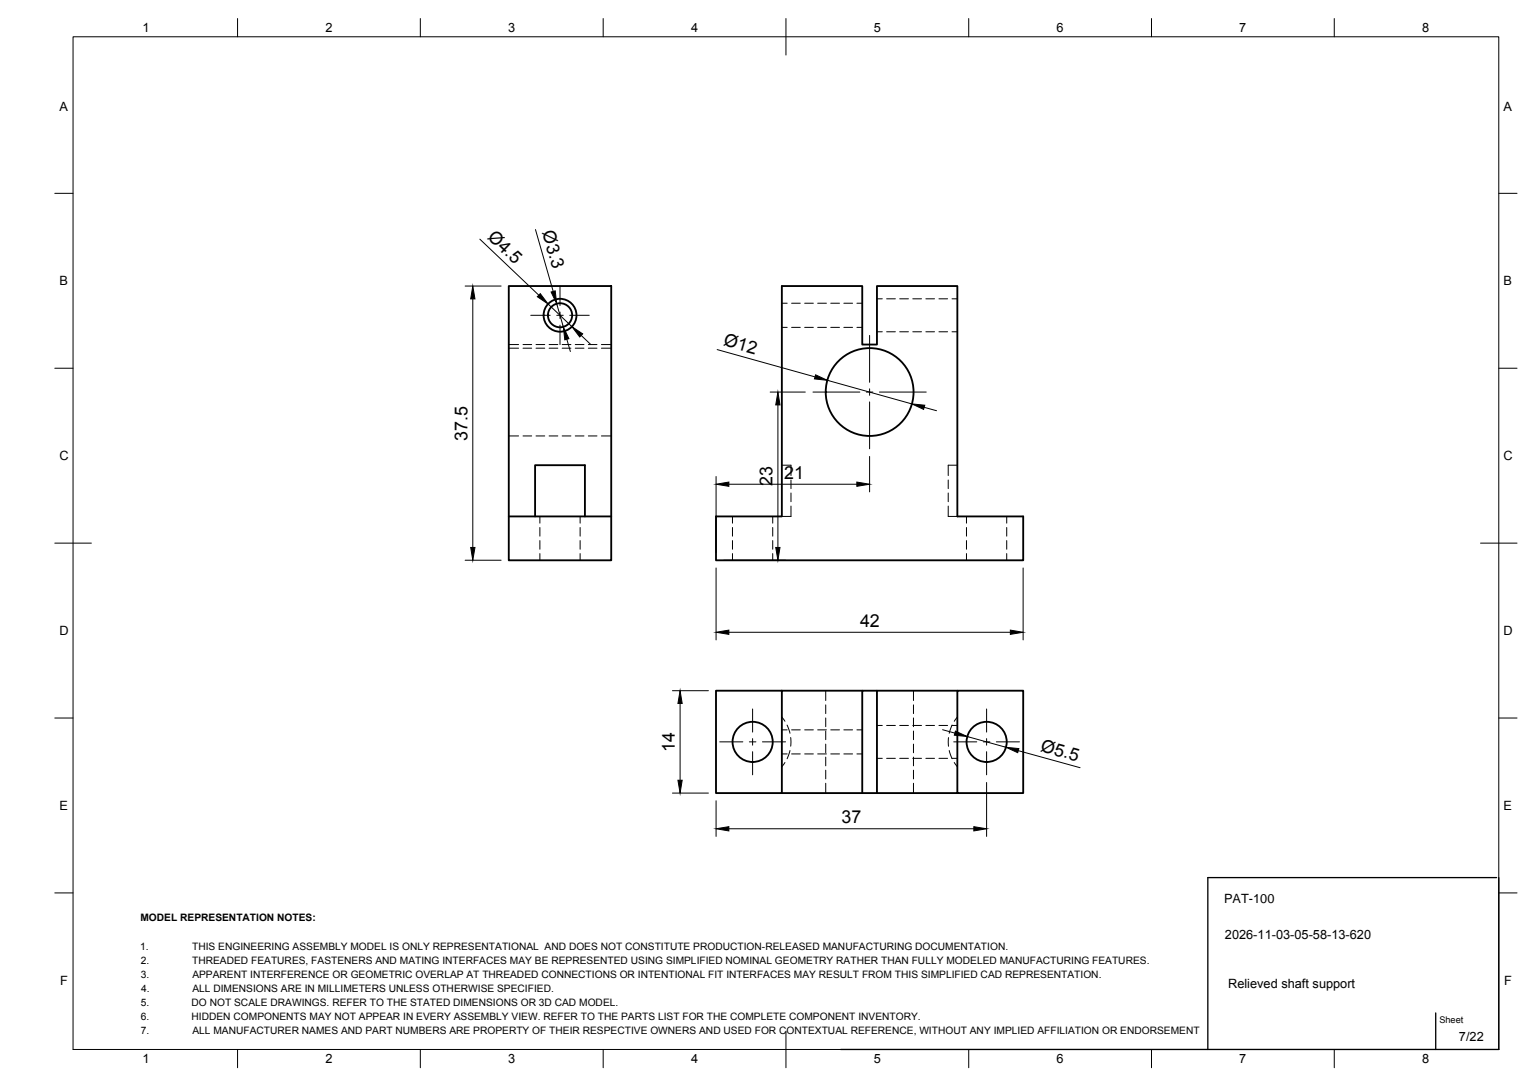
ISO-10303-21;
HEADER;
/* Generated by software containing ST-Developer
 * from STEP Tools, Inc. (www.steptools.com) 
 */

FILE_DESCRIPTION(
/* description */ (''),
/* implementation_level */ '2;1');

FILE_NAME(
/* name */ 'Relieved shaft support.step',
/* time_stamp */ '2026-10-29T16:43:51-07:00',
/* author */ (''),
/* organization */ (''),
/* preprocessor_version */ 'ST-DEVELOPER v20.2',
/* originating_system */ 'Autodesk Translation Framework v15.17.0.0',
/* authorisation */ '');

FILE_SCHEMA (('AUTOMOTIVE_DESIGN { 1 0 10303 214 3 1 1 }'));
ENDSEC;

DATA;
#10=MECHANICAL_DESIGN_GEOMETRIC_PRESENTATION_REPRESENTATION('',(#367),#10292);
#321=SHAPE_REPRESENTATION_RELATIONSHIP('SRR','None',#10417,#344);
#344=ADVANCED_BREP_SHAPE_REPRESENTATION('',(#390),#10269);
#367=STYLED_ITEM('',(#10628),#390);
#390=MANIFOLD_SOLID_BREP('Body1',#5009);
#438=FACE_BOUND('',#1062,.T.);
#439=FACE_BOUND('',#1064,.T.);
#440=FACE_BOUND('',#1066,.T.);
#441=FACE_BOUND('',#1073,.T.);
#442=FACE_BOUND('',#1076,.T.);
#443=FACE_BOUND('',#1077,.T.);
#444=FACE_BOUND('',#1080,.T.);
#445=FACE_BOUND('',#1083,.T.);
#446=FACE_BOUND('',#1086,.T.);
#447=FACE_BOUND('',#1089,.T.);
#539=PLANE('',#5357);
#540=PLANE('',#5364);
#541=PLANE('',#5365);
#542=PLANE('',#5367);
#543=PLANE('',#5369);
#544=PLANE('',#5383);
#545=PLANE('',#5384);
#546=PLANE('',#5385);
#547=PLANE('',#5386);
#548=PLANE('',#5387);
#549=PLANE('',#5388);
#550=PLANE('',#5389);
#551=PLANE('',#5390);
#552=PLANE('',#5391);
#553=PLANE('',#5392);
#554=PLANE('',#5393);
#737=FACE_OUTER_BOUND('',#1057,.T.);
#738=FACE_OUTER_BOUND('',#1058,.T.);
#739=FACE_OUTER_BOUND('',#1059,.T.);
#740=FACE_OUTER_BOUND('',#1060,.T.);
#741=FACE_OUTER_BOUND('',#1061,.T.);
#742=FACE_OUTER_BOUND('',#1063,.T.);
#743=FACE_OUTER_BOUND('',#1065,.T.);
#744=FACE_OUTER_BOUND('',#1067,.T.);
#745=FACE_OUTER_BOUND('',#1068,.T.);
#746=FACE_OUTER_BOUND('',#1069,.T.);
#747=FACE_OUTER_BOUND('',#1070,.T.);
#748=FACE_OUTER_BOUND('',#1071,.T.);
#749=FACE_OUTER_BOUND('',#1072,.T.);
#750=FACE_OUTER_BOUND('',#1074,.T.);
#751=FACE_OUTER_BOUND('',#1075,.T.);
#752=FACE_OUTER_BOUND('',#1078,.T.);
#753=FACE_OUTER_BOUND('',#1079,.T.);
#754=FACE_OUTER_BOUND('',#1081,.T.);
#755=FACE_OUTER_BOUND('',#1082,.T.);
#756=FACE_OUTER_BOUND('',#1084,.T.);
#757=FACE_OUTER_BOUND('',#1085,.T.);
#758=FACE_OUTER_BOUND('',#1087,.T.);
#759=FACE_OUTER_BOUND('',#1088,.T.);
#1057=EDGE_LOOP('',(#3543,#3544));
#1058=EDGE_LOOP('',(#3545,#3546,#3547,#3548));
#1059=EDGE_LOOP('',(#3549,#3550,#3551,#3552));
#1060=EDGE_LOOP('',(#3553,#3554));
#1061=EDGE_LOOP('',(#3555,#3556,#3557,#3558,#3559,#3560));
#1062=EDGE_LOOP('',(#3561));
#1063=EDGE_LOOP('',(#3562,#3563,#3564,#3565,#3566,#3567,#3568,#3569));
#1064=EDGE_LOOP('',(#3570));
#1065=EDGE_LOOP('',(#3571,#3572,#3573,#3574,#3575,#3576));
#1066=EDGE_LOOP('',(#3577));
#1067=EDGE_LOOP('',(#3578,#3579,#3580,#3581));
#1068=EDGE_LOOP('',(#3582,#3583,#3584,#3585));
#1069=EDGE_LOOP('',(#3586,#3587,#3588,#3589));
#1070=EDGE_LOOP('',(#3590,#3591,#3592,#3593));
#1071=EDGE_LOOP('',(#3594,#3595,#3596,#3597));
#1072=EDGE_LOOP('',(#3598,#3599,#3600,#3601,#3602,#3603,#3604,#3605,#3606,
#3607,#3608,#3609));
#1073=EDGE_LOOP('',(#3610));
#1074=EDGE_LOOP('',(#3611,#3612,#3613,#3614));
#1075=EDGE_LOOP('',(#3615,#3616,#3617,#3618));
#1076=EDGE_LOOP('',(#3619));
#1077=EDGE_LOOP('',(#3620));
#1078=EDGE_LOOP('',(#3621,#3622,#3623,#3624));
#1079=EDGE_LOOP('',(#3625,#3626,#3627,#3628,#3629,#3630,#3631,#3632));
#1080=EDGE_LOOP('',(#3633));
#1081=EDGE_LOOP('',(#3634,#3635,#3636,#3637));
#1082=EDGE_LOOP('',(#3638,#3639,#3640,#3641));
#1083=EDGE_LOOP('',(#3642));
#1084=EDGE_LOOP('',(#3643,#3644,#3645,#3646));
#1085=EDGE_LOOP('',(#3647,#3648,#3649,#3650));
#1086=EDGE_LOOP('',(#3651));
#1087=EDGE_LOOP('',(#3652,#3653,#3654,#3655));
#1088=EDGE_LOOP('',(#3656,#3657,#3658,#3659,#3660,#3661,#3662,#3663,#3664,
#3665,#3666,#3667));
#1089=EDGE_LOOP('',(#3668));
#1442=LINE('',#7552,#1834);
#1443=LINE('',#7556,#1835);
#1444=LINE('',#7559,#1836);
#1445=LINE('',#7563,#1837);
#1446=LINE('',#7567,#1838);
#1447=LINE('',#7570,#1839);
#1448=LINE('',#7573,#1840);
#1449=LINE('',#7575,#1841);
#1450=LINE('',#7577,#1842);
#1451=LINE('',#7579,#1843);
#1452=LINE('',#7580,#1844);
#1453=LINE('',#7585,#1845);
#1454=LINE('',#7587,#1846);
#1455=LINE('',#7588,#1847);
#1456=LINE('',#7594,#1848);
#1457=LINE('',#7596,#1849);
#1458=LINE('',#7597,#1850);
#1459=LINE('',#7599,#1851);
#1460=LINE('',#7600,#1852);
#1461=LINE('',#7607,#1853);
#1462=LINE('',#7611,#1854);
#1463=LINE('',#7616,#1855);
#1464=LINE('',#7620,#1856);
#1465=LINE('',#7625,#1857);
#1466=LINE('',#7629,#1858);
#1467=LINE('',#7631,#1859);
#1468=LINE('',#7632,#1860);
#1469=LINE('',#7634,#1861);
#1470=LINE('',#7636,#1862);
#1471=LINE('',#7638,#1863);
#1472=LINE('',#7640,#1864);
#1473=LINE('',#7642,#1865);
#1474=LINE('',#7643,#1866);
#1475=LINE('',#7646,#1867);
#1476=LINE('',#7647,#1868);
#1477=LINE('',#7650,#1869);
#1478=LINE('',#7651,#1870);
#1479=LINE('',#7653,#1871);
#1480=LINE('',#7656,#1872);
#1481=LINE('',#7657,#1873);
#1482=LINE('',#7660,#1874);
#1483=LINE('',#7661,#1875);
#1484=LINE('',#7664,#1876);
#1485=LINE('',#7665,#1877);
#1486=LINE('',#7668,#1878);
#1487=LINE('',#7669,#1879);
#1488=LINE('',#7672,#1880);
#1489=LINE('',#7673,#1881);
#1490=LINE('',#7675,#1882);
#1834=VECTOR('',#6033,1.);
#1835=VECTOR('',#6038,1.);
#1836=VECTOR('',#6041,1.);
#1837=VECTOR('',#6044,1.);
#1838=VECTOR('',#6047,1.);
#1839=VECTOR('',#6052,1.);
#1840=VECTOR('',#6055,1.);
#1841=VECTOR('',#6056,1.);
#1842=VECTOR('',#6057,1.);
#1843=VECTOR('',#6058,1.);
#1844=VECTOR('',#6059,1.);
#1845=VECTOR('',#6064,1.);
#1846=VECTOR('',#6065,1.);
#1847=VECTOR('',#6066,1.);
#1848=VECTOR('',#6071,1.);
#1849=VECTOR('',#6072,1.);
#1850=VECTOR('',#6073,1.);
#1851=VECTOR('',#6074,1.);
#1852=VECTOR('',#6075,1.);
#1853=VECTOR('',#6082,0.225);
#1854=VECTOR('',#6087,0.165);
#1855=VECTOR('',#6094,0.275);
#1856=VECTOR('',#6099,0.275);
#1857=VECTOR('',#6104,0.6);
#1858=VECTOR('',#6109,1.);
#1859=VECTOR('',#6110,1.);
#1860=VECTOR('',#6111,1.);
#1861=VECTOR('',#6112,1.);
#1862=VECTOR('',#6113,1.);
#1863=VECTOR('',#6114,1.);
#1864=VECTOR('',#6115,1.);
#1865=VECTOR('',#6116,1.);
#1866=VECTOR('',#6117,1.);
#1867=VECTOR('',#6120,1.);
#1868=VECTOR('',#6121,1.);
#1869=VECTOR('',#6124,1.);
#1870=VECTOR('',#6125,1.);
#1871=VECTOR('',#6128,1.);
#1872=VECTOR('',#6131,1.);
#1873=VECTOR('',#6132,1.);
#1874=VECTOR('',#6135,1.);
#1875=VECTOR('',#6136,1.);
#1876=VECTOR('',#6139,1.);
#1877=VECTOR('',#6140,1.);
#1878=VECTOR('',#6143,1.);
#1879=VECTOR('',#6144,1.);
#1880=VECTOR('',#6147,1.);
#1881=VECTOR('',#6148,1.);
#1882=VECTOR('',#6151,1.);
#2231=CIRCLE('',#5358,0.525);
#2232=CIRCLE('',#5360,0.525);
#2233=CIRCLE('',#5362,0.525);
#2234=CIRCLE('',#5363,0.525);
#2235=CIRCLE('',#5366,0.275);
#2236=CIRCLE('',#5368,0.165);
#2237=CIRCLE('',#5370,0.275);
#2238=CIRCLE('',#5372,0.225);
#2239=CIRCLE('',#5373,0.225);
#2240=CIRCLE('',#5375,0.165);
#2241=CIRCLE('',#5377,0.275);
#2242=CIRCLE('',#5379,0.275);
#2243=CIRCLE('',#5381,0.6);
#2244=CIRCLE('',#5382,0.6);
#2438=VERTEX_POINT('',#7550);
#2439=VERTEX_POINT('',#7551);
#2440=VERTEX_POINT('',#7555);
#2441=VERTEX_POINT('',#7557);
#2442=VERTEX_POINT('',#7561);
#2443=VERTEX_POINT('',#7562);
#2444=VERTEX_POINT('',#7564);
#2445=VERTEX_POINT('',#7566);
#2446=VERTEX_POINT('',#7572);
#2447=VERTEX_POINT('',#7574);
#2448=VERTEX_POINT('',#7576);
#2449=VERTEX_POINT('',#7578);
#2450=VERTEX_POINT('',#7581);
#2451=VERTEX_POINT('',#7584);
#2452=VERTEX_POINT('',#7586);
#2453=VERTEX_POINT('',#7589);
#2454=VERTEX_POINT('',#7592);
#2455=VERTEX_POINT('',#7593);
#2456=VERTEX_POINT('',#7595);
#2457=VERTEX_POINT('',#7598);
#2458=VERTEX_POINT('',#7601);
#2459=VERTEX_POINT('',#7604);
#2460=VERTEX_POINT('',#7606);
#2461=VERTEX_POINT('',#7610);
#2462=VERTEX_POINT('',#7614);
#2463=VERTEX_POINT('',#7618);
#2464=VERTEX_POINT('',#7622);
#2465=VERTEX_POINT('',#7624);
#2466=VERTEX_POINT('',#7628);
#2467=VERTEX_POINT('',#7630);
#2468=VERTEX_POINT('',#7633);
#2469=VERTEX_POINT('',#7635);
#2470=VERTEX_POINT('',#7637);
#2471=VERTEX_POINT('',#7639);
#2472=VERTEX_POINT('',#7641);
#2473=VERTEX_POINT('',#7645);
#2474=VERTEX_POINT('',#7649);
#2475=VERTEX_POINT('',#7655);
#2476=VERTEX_POINT('',#7659);
#2477=VERTEX_POINT('',#7663);
#2478=VERTEX_POINT('',#7667);
#2479=VERTEX_POINT('',#7671);
#2862=EDGE_CURVE('',#2438,#2439,#1442,.T.);
#2863=EDGE_CURVE('',#2439,#2438,#2231,.T.);
#2864=EDGE_CURVE('',#2440,#2438,#1443,.T.);
#2865=EDGE_CURVE('',#2441,#2440,#2232,.T.);
#2866=EDGE_CURVE('',#2439,#2441,#1444,.T.);
#2867=EDGE_CURVE('',#2442,#2443,#1445,.T.);
#2868=EDGE_CURVE('',#2442,#2444,#2233,.T.);
#2869=EDGE_CURVE('',#2445,#2444,#1446,.T.);
#2870=EDGE_CURVE('',#2443,#2445,#2234,.T.);
#2871=EDGE_CURVE('',#2444,#2442,#1447,.T.);
#2872=EDGE_CURVE('',#2440,#2446,#1448,.T.);
#2873=EDGE_CURVE('',#2447,#2446,#1449,.T.);
#2874=EDGE_CURVE('',#2447,#2448,#1450,.T.);
#2875=EDGE_CURVE('',#2449,#2448,#1451,.T.);
#2876=EDGE_CURVE('',#2449,#2441,#1452,.T.);
#2877=EDGE_CURVE('',#2450,#2450,#2235,.T.);
#2878=EDGE_CURVE('',#2451,#2449,#1453,.T.);
#2879=EDGE_CURVE('',#2451,#2452,#1454,.T.);
#2880=EDGE_CURVE('',#2446,#2452,#1455,.T.);
#2881=EDGE_CURVE('',#2453,#2453,#2236,.T.);
#2882=EDGE_CURVE('',#2454,#2455,#1456,.T.);
#2883=EDGE_CURVE('',#2456,#2455,#1457,.T.);
#2884=EDGE_CURVE('',#2443,#2456,#1458,.T.);
#2885=EDGE_CURVE('',#2457,#2445,#1459,.T.);
#2886=EDGE_CURVE('',#2454,#2457,#1460,.T.);
#2887=EDGE_CURVE('',#2458,#2458,#2237,.T.);
#2888=EDGE_CURVE('',#2459,#2459,#2238,.T.);
#2889=EDGE_CURVE('',#2459,#2460,#1461,.T.);
#2890=EDGE_CURVE('',#2460,#2460,#2239,.T.);
#2891=EDGE_CURVE('',#2453,#2461,#1462,.T.);
#2892=EDGE_CURVE('',#2461,#2461,#2240,.T.);
#2893=EDGE_CURVE('',#2462,#2462,#2241,.T.);
#2894=EDGE_CURVE('',#2462,#2450,#1463,.T.);
#2895=EDGE_CURVE('',#2463,#2463,#2242,.T.);
#2896=EDGE_CURVE('',#2463,#2458,#1464,.T.);
#2897=EDGE_CURVE('',#2464,#2464,#2243,.T.);
#2898=EDGE_CURVE('',#2464,#2465,#1465,.T.);
#2899=EDGE_CURVE('',#2465,#2465,#2244,.T.);
#2900=EDGE_CURVE('',#2448,#2466,#1466,.T.);
#2901=EDGE_CURVE('',#2466,#2467,#1467,.T.);
#2902=EDGE_CURVE('',#2467,#2454,#1468,.T.);
#2903=EDGE_CURVE('',#2457,#2468,#1469,.T.);
#2904=EDGE_CURVE('',#2468,#2469,#1470,.T.);
#2905=EDGE_CURVE('',#2469,#2470,#1471,.T.);
#2906=EDGE_CURVE('',#2470,#2471,#1472,.T.);
#2907=EDGE_CURVE('',#2471,#2472,#1473,.T.);
#2908=EDGE_CURVE('',#2472,#2451,#1474,.T.);
#2909=EDGE_CURVE('',#2473,#2447,#1475,.T.);
#2910=EDGE_CURVE('',#2466,#2473,#1476,.T.);
#2911=EDGE_CURVE('',#2474,#2473,#1477,.T.);
#2912=EDGE_CURVE('',#2467,#2474,#1478,.T.);
#2913=EDGE_CURVE('',#2455,#2474,#1479,.T.);
#2914=EDGE_CURVE('',#2475,#2456,#1480,.T.);
#2915=EDGE_CURVE('',#2468,#2475,#1481,.T.);
#2916=EDGE_CURVE('',#2476,#2475,#1482,.T.);
#2917=EDGE_CURVE('',#2469,#2476,#1483,.T.);
#2918=EDGE_CURVE('',#2477,#2476,#1484,.T.);
#2919=EDGE_CURVE('',#2470,#2477,#1485,.T.);
#2920=EDGE_CURVE('',#2478,#2477,#1486,.T.);
#2921=EDGE_CURVE('',#2471,#2478,#1487,.T.);
#2922=EDGE_CURVE('',#2479,#2478,#1488,.T.);
#2923=EDGE_CURVE('',#2472,#2479,#1489,.T.);
#2924=EDGE_CURVE('',#2452,#2479,#1490,.T.);
#3543=ORIENTED_EDGE('',*,*,#2862,.F.);
#3544=ORIENTED_EDGE('',*,*,#2863,.F.);
#3545=ORIENTED_EDGE('',*,*,#2864,.F.);
#3546=ORIENTED_EDGE('',*,*,#2865,.F.);
#3547=ORIENTED_EDGE('',*,*,#2866,.F.);
#3548=ORIENTED_EDGE('',*,*,#2863,.T.);
#3549=ORIENTED_EDGE('',*,*,#2867,.F.);
#3550=ORIENTED_EDGE('',*,*,#2868,.T.);
#3551=ORIENTED_EDGE('',*,*,#2869,.F.);
#3552=ORIENTED_EDGE('',*,*,#2870,.F.);
#3553=ORIENTED_EDGE('',*,*,#2871,.F.);
#3554=ORIENTED_EDGE('',*,*,#2868,.F.);
#3555=ORIENTED_EDGE('',*,*,#2872,.T.);
#3556=ORIENTED_EDGE('',*,*,#2873,.F.);
#3557=ORIENTED_EDGE('',*,*,#2874,.T.);
#3558=ORIENTED_EDGE('',*,*,#2875,.F.);
#3559=ORIENTED_EDGE('',*,*,#2876,.T.);
#3560=ORIENTED_EDGE('',*,*,#2865,.T.);
#3561=ORIENTED_EDGE('',*,*,#2877,.T.);
#3562=ORIENTED_EDGE('',*,*,#2864,.T.);
#3563=ORIENTED_EDGE('',*,*,#2862,.T.);
#3564=ORIENTED_EDGE('',*,*,#2866,.T.);
#3565=ORIENTED_EDGE('',*,*,#2876,.F.);
#3566=ORIENTED_EDGE('',*,*,#2878,.F.);
#3567=ORIENTED_EDGE('',*,*,#2879,.T.);
#3568=ORIENTED_EDGE('',*,*,#2880,.F.);
#3569=ORIENTED_EDGE('',*,*,#2872,.F.);
#3570=ORIENTED_EDGE('',*,*,#2881,.T.);
#3571=ORIENTED_EDGE('',*,*,#2882,.T.);
#3572=ORIENTED_EDGE('',*,*,#2883,.F.);
#3573=ORIENTED_EDGE('',*,*,#2884,.F.);
#3574=ORIENTED_EDGE('',*,*,#2870,.T.);
#3575=ORIENTED_EDGE('',*,*,#2885,.F.);
#3576=ORIENTED_EDGE('',*,*,#2886,.F.);
#3577=ORIENTED_EDGE('',*,*,#2887,.T.);
#3578=ORIENTED_EDGE('',*,*,#2888,.F.);
#3579=ORIENTED_EDGE('',*,*,#2889,.T.);
#3580=ORIENTED_EDGE('',*,*,#2890,.F.);
#3581=ORIENTED_EDGE('',*,*,#2889,.F.);
#3582=ORIENTED_EDGE('',*,*,#2881,.F.);
#3583=ORIENTED_EDGE('',*,*,#2891,.T.);
#3584=ORIENTED_EDGE('',*,*,#2892,.F.);
#3585=ORIENTED_EDGE('',*,*,#2891,.F.);
#3586=ORIENTED_EDGE('',*,*,#2893,.F.);
#3587=ORIENTED_EDGE('',*,*,#2894,.T.);
#3588=ORIENTED_EDGE('',*,*,#2877,.F.);
#3589=ORIENTED_EDGE('',*,*,#2894,.F.);
#3590=ORIENTED_EDGE('',*,*,#2895,.F.);
#3591=ORIENTED_EDGE('',*,*,#2896,.T.);
#3592=ORIENTED_EDGE('',*,*,#2887,.F.);
#3593=ORIENTED_EDGE('',*,*,#2896,.F.);
#3594=ORIENTED_EDGE('',*,*,#2897,.F.);
#3595=ORIENTED_EDGE('',*,*,#2898,.T.);
#3596=ORIENTED_EDGE('',*,*,#2899,.F.);
#3597=ORIENTED_EDGE('',*,*,#2898,.F.);
#3598=ORIENTED_EDGE('',*,*,#2875,.T.);
#3599=ORIENTED_EDGE('',*,*,#2900,.T.);
#3600=ORIENTED_EDGE('',*,*,#2901,.T.);
#3601=ORIENTED_EDGE('',*,*,#2902,.T.);
#3602=ORIENTED_EDGE('',*,*,#2886,.T.);
#3603=ORIENTED_EDGE('',*,*,#2903,.T.);
#3604=ORIENTED_EDGE('',*,*,#2904,.T.);
#3605=ORIENTED_EDGE('',*,*,#2905,.T.);
#3606=ORIENTED_EDGE('',*,*,#2906,.T.);
#3607=ORIENTED_EDGE('',*,*,#2907,.T.);
#3608=ORIENTED_EDGE('',*,*,#2908,.T.);
#3609=ORIENTED_EDGE('',*,*,#2878,.T.);
#3610=ORIENTED_EDGE('',*,*,#2897,.T.);
#3611=ORIENTED_EDGE('',*,*,#2874,.F.);
#3612=ORIENTED_EDGE('',*,*,#2909,.F.);
#3613=ORIENTED_EDGE('',*,*,#2910,.F.);
#3614=ORIENTED_EDGE('',*,*,#2900,.F.);
#3615=ORIENTED_EDGE('',*,*,#2910,.T.);
#3616=ORIENTED_EDGE('',*,*,#2911,.F.);
#3617=ORIENTED_EDGE('',*,*,#2912,.F.);
#3618=ORIENTED_EDGE('',*,*,#2901,.F.);
#3619=ORIENTED_EDGE('',*,*,#2893,.T.);
#3620=ORIENTED_EDGE('',*,*,#2895,.T.);
#3621=ORIENTED_EDGE('',*,*,#2912,.T.);
#3622=ORIENTED_EDGE('',*,*,#2913,.F.);
#3623=ORIENTED_EDGE('',*,*,#2882,.F.);
#3624=ORIENTED_EDGE('',*,*,#2902,.F.);
#3625=ORIENTED_EDGE('',*,*,#2867,.T.);
#3626=ORIENTED_EDGE('',*,*,#2884,.T.);
#3627=ORIENTED_EDGE('',*,*,#2914,.F.);
#3628=ORIENTED_EDGE('',*,*,#2915,.F.);
#3629=ORIENTED_EDGE('',*,*,#2903,.F.);
#3630=ORIENTED_EDGE('',*,*,#2885,.T.);
#3631=ORIENTED_EDGE('',*,*,#2869,.T.);
#3632=ORIENTED_EDGE('',*,*,#2871,.T.);
#3633=ORIENTED_EDGE('',*,*,#2890,.T.);
#3634=ORIENTED_EDGE('',*,*,#2915,.T.);
#3635=ORIENTED_EDGE('',*,*,#2916,.F.);
#3636=ORIENTED_EDGE('',*,*,#2917,.F.);
#3637=ORIENTED_EDGE('',*,*,#2904,.F.);
#3638=ORIENTED_EDGE('',*,*,#2917,.T.);
#3639=ORIENTED_EDGE('',*,*,#2918,.F.);
#3640=ORIENTED_EDGE('',*,*,#2919,.F.);
#3641=ORIENTED_EDGE('',*,*,#2905,.F.);
#3642=ORIENTED_EDGE('',*,*,#2888,.T.);
#3643=ORIENTED_EDGE('',*,*,#2919,.T.);
#3644=ORIENTED_EDGE('',*,*,#2920,.F.);
#3645=ORIENTED_EDGE('',*,*,#2921,.F.);
#3646=ORIENTED_EDGE('',*,*,#2906,.F.);
#3647=ORIENTED_EDGE('',*,*,#2921,.T.);
#3648=ORIENTED_EDGE('',*,*,#2922,.F.);
#3649=ORIENTED_EDGE('',*,*,#2923,.F.);
#3650=ORIENTED_EDGE('',*,*,#2907,.F.);
#3651=ORIENTED_EDGE('',*,*,#2892,.T.);
#3652=ORIENTED_EDGE('',*,*,#2923,.T.);
#3653=ORIENTED_EDGE('',*,*,#2924,.F.);
#3654=ORIENTED_EDGE('',*,*,#2879,.F.);
#3655=ORIENTED_EDGE('',*,*,#2908,.F.);
#3656=ORIENTED_EDGE('',*,*,#2873,.T.);
#3657=ORIENTED_EDGE('',*,*,#2880,.T.);
#3658=ORIENTED_EDGE('',*,*,#2924,.T.);
#3659=ORIENTED_EDGE('',*,*,#2922,.T.);
#3660=ORIENTED_EDGE('',*,*,#2920,.T.);
#3661=ORIENTED_EDGE('',*,*,#2918,.T.);
#3662=ORIENTED_EDGE('',*,*,#2916,.T.);
#3663=ORIENTED_EDGE('',*,*,#2914,.T.);
#3664=ORIENTED_EDGE('',*,*,#2883,.T.);
#3665=ORIENTED_EDGE('',*,*,#2913,.T.);
#3666=ORIENTED_EDGE('',*,*,#2911,.T.);
#3667=ORIENTED_EDGE('',*,*,#2909,.T.);
#3668=ORIENTED_EDGE('',*,*,#2899,.T.);
#4654=CYLINDRICAL_SURFACE('',#5359,0.525);
#4655=CYLINDRICAL_SURFACE('',#5361,0.525);
#4656=CYLINDRICAL_SURFACE('',#5371,0.225);
#4657=CYLINDRICAL_SURFACE('',#5374,0.165);
#4658=CYLINDRICAL_SURFACE('',#5376,0.275);
#4659=CYLINDRICAL_SURFACE('',#5378,0.275);
#4660=CYLINDRICAL_SURFACE('',#5380,0.6);
#4746=ADVANCED_FACE('',(#737),#539,.F.);
#4747=ADVANCED_FACE('',(#738),#4654,.F.);
#4748=ADVANCED_FACE('',(#739),#4655,.F.);
#4749=ADVANCED_FACE('',(#740),#540,.F.);
#4750=ADVANCED_FACE('',(#741,#438),#541,.T.);
#4751=ADVANCED_FACE('',(#742,#439),#542,.T.);
#4752=ADVANCED_FACE('',(#743,#440),#543,.T.);
#4753=ADVANCED_FACE('',(#744),#4656,.F.);
#4754=ADVANCED_FACE('',(#745),#4657,.F.);
#4755=ADVANCED_FACE('',(#746),#4658,.F.);
#4756=ADVANCED_FACE('',(#747),#4659,.F.);
#4757=ADVANCED_FACE('',(#748),#4660,.F.);
#4758=ADVANCED_FACE('',(#749,#441),#544,.T.);
#4759=ADVANCED_FACE('',(#750),#545,.T.);
#4760=ADVANCED_FACE('',(#751,#442,#443),#546,.T.);
#4761=ADVANCED_FACE('',(#752),#547,.T.);
#4762=ADVANCED_FACE('',(#753,#444),#548,.T.);
#4763=ADVANCED_FACE('',(#754),#549,.T.);
#4764=ADVANCED_FACE('',(#755,#445),#550,.T.);
#4765=ADVANCED_FACE('',(#756),#551,.T.);
#4766=ADVANCED_FACE('',(#757,#446),#552,.T.);
#4767=ADVANCED_FACE('',(#758),#553,.T.);
#4768=ADVANCED_FACE('',(#759,#447),#554,.T.);
#5009=CLOSED_SHELL('',(#4746,#4747,#4748,#4749,#4750,#4751,#4752,#4753,
#4754,#4755,#4756,#4757,#4758,#4759,#4760,#4761,#4762,#4763,#4764,#4765,
#4766,#4767,#4768));
#5356=AXIS2_PLACEMENT_3D('',#7548,#6029,#6030);
#5357=AXIS2_PLACEMENT_3D('',#7549,#6031,#6032);
#5358=AXIS2_PLACEMENT_3D('',#7553,#6034,#6035);
#5359=AXIS2_PLACEMENT_3D('',#7554,#6036,#6037);
#5360=AXIS2_PLACEMENT_3D('',#7558,#6039,#6040);
#5361=AXIS2_PLACEMENT_3D('',#7560,#6042,#6043);
#5362=AXIS2_PLACEMENT_3D('',#7565,#6045,#6046);
#5363=AXIS2_PLACEMENT_3D('',#7568,#6048,#6049);
#5364=AXIS2_PLACEMENT_3D('',#7569,#6050,#6051);
#5365=AXIS2_PLACEMENT_3D('',#7571,#6053,#6054);
#5366=AXIS2_PLACEMENT_3D('',#7582,#6060,#6061);
#5367=AXIS2_PLACEMENT_3D('',#7583,#6062,#6063);
#5368=AXIS2_PLACEMENT_3D('',#7590,#6067,#6068);
#5369=AXIS2_PLACEMENT_3D('',#7591,#6069,#6070);
#5370=AXIS2_PLACEMENT_3D('',#7602,#6076,#6077);
#5371=AXIS2_PLACEMENT_3D('',#7603,#6078,#6079);
#5372=AXIS2_PLACEMENT_3D('',#7605,#6080,#6081);
#5373=AXIS2_PLACEMENT_3D('',#7608,#6083,#6084);
#5374=AXIS2_PLACEMENT_3D('',#7609,#6085,#6086);
#5375=AXIS2_PLACEMENT_3D('',#7612,#6088,#6089);
#5376=AXIS2_PLACEMENT_3D('',#7613,#6090,#6091);
#5377=AXIS2_PLACEMENT_3D('',#7615,#6092,#6093);
#5378=AXIS2_PLACEMENT_3D('',#7617,#6095,#6096);
#5379=AXIS2_PLACEMENT_3D('',#7619,#6097,#6098);
#5380=AXIS2_PLACEMENT_3D('',#7621,#6100,#6101);
#5381=AXIS2_PLACEMENT_3D('',#7623,#6102,#6103);
#5382=AXIS2_PLACEMENT_3D('',#7626,#6105,#6106);
#5383=AXIS2_PLACEMENT_3D('',#7627,#6107,#6108);
#5384=AXIS2_PLACEMENT_3D('',#7644,#6118,#6119);
#5385=AXIS2_PLACEMENT_3D('',#7648,#6122,#6123);
#5386=AXIS2_PLACEMENT_3D('',#7652,#6126,#6127);
#5387=AXIS2_PLACEMENT_3D('',#7654,#6129,#6130);
#5388=AXIS2_PLACEMENT_3D('',#7658,#6133,#6134);
#5389=AXIS2_PLACEMENT_3D('',#7662,#6137,#6138);
#5390=AXIS2_PLACEMENT_3D('',#7666,#6141,#6142);
#5391=AXIS2_PLACEMENT_3D('',#7670,#6145,#6146);
#5392=AXIS2_PLACEMENT_3D('',#7674,#6149,#6150);
#5393=AXIS2_PLACEMENT_3D('',#7676,#6152,#6153);
#6029=DIRECTION('axis',(0.,0.,1.));
#6030=DIRECTION('refdir',(1.,0.,0.));
#6031=DIRECTION('center_axis',(0.,0.,1.));
#6032=DIRECTION('ref_axis',(1.,0.,0.));
#6033=DIRECTION('',(0.,-1.,0.));
#6034=DIRECTION('center_axis',(0.,0.,1.));
#6035=DIRECTION('ref_axis',(1.,0.,0.));
#6036=DIRECTION('center_axis',(0.,0.,1.));
#6037=DIRECTION('ref_axis',(1.,0.,0.));
#6038=DIRECTION('',(0.,0.,1.));
#6039=DIRECTION('center_axis',(0.,0.,1.));
#6040=DIRECTION('ref_axis',(1.,0.,0.));
#6041=DIRECTION('',(0.,0.,-1.));
#6042=DIRECTION('center_axis',(0.,0.,1.));
#6043=DIRECTION('ref_axis',(-1.,1.22464679914735E-16,0.));
#6044=DIRECTION('',(0.,0.,-1.));
#6045=DIRECTION('center_axis',(0.,0.,1.));
#6046=DIRECTION('ref_axis',(1.,0.,0.));
#6047=DIRECTION('',(0.,0.,1.));
#6048=DIRECTION('center_axis',(0.,0.,1.));
#6049=DIRECTION('ref_axis',(1.,0.,0.));
#6050=DIRECTION('center_axis',(0.,0.,1.));
#6051=DIRECTION('ref_axis',(1.,0.,0.));
#6052=DIRECTION('',(0.,1.,0.));
#6053=DIRECTION('center_axis',(0.,0.,1.));
#6054=DIRECTION('ref_axis',(1.,0.,0.));
#6055=DIRECTION('',(0.,1.,0.));
#6056=DIRECTION('',(1.,0.,0.));
#6057=DIRECTION('',(0.,-1.,0.));
#6058=DIRECTION('',(-1.,0.,0.));
#6059=DIRECTION('',(0.,1.,0.));
#6060=DIRECTION('center_axis',(0.,0.,-1.));
#6061=DIRECTION('ref_axis',(1.,0.,0.));
#6062=DIRECTION('center_axis',(-1.,0.,0.));
#6063=DIRECTION('ref_axis',(0.,0.,1.));
#6064=DIRECTION('',(0.,0.,-1.));
#6065=DIRECTION('',(0.,1.,0.));
#6066=DIRECTION('',(0.,0.,1.));
#6067=DIRECTION('center_axis',(1.,0.,0.));
#6068=DIRECTION('ref_axis',(0.,0.,-1.));
#6069=DIRECTION('center_axis',(0.,0.,1.));
#6070=DIRECTION('ref_axis',(1.,0.,0.));
#6071=DIRECTION('',(0.,1.,0.));
#6072=DIRECTION('',(1.,0.,0.));
#6073=DIRECTION('',(0.,1.,0.));
#6074=DIRECTION('',(0.,1.,0.));
#6075=DIRECTION('',(-1.,0.,0.));
#6076=DIRECTION('center_axis',(0.,0.,-1.));
#6077=DIRECTION('ref_axis',(1.,0.,0.));
#6078=DIRECTION('center_axis',(1.,0.,0.));
#6079=DIRECTION('ref_axis',(0.,0.,-1.));
#6080=DIRECTION('center_axis',(1.,0.,0.));
#6081=DIRECTION('ref_axis',(0.,0.,-1.));
#6082=DIRECTION('',(1.,0.,0.));
#6083=DIRECTION('center_axis',(-1.,0.,0.));
#6084=DIRECTION('ref_axis',(0.,0.,-1.));
#6085=DIRECTION('center_axis',(1.,0.,0.));
#6086=DIRECTION('ref_axis',(0.,0.,-1.));
#6087=DIRECTION('',(1.,0.,0.));
#6088=DIRECTION('center_axis',(-1.,0.,0.));
#6089=DIRECTION('ref_axis',(0.,0.,-1.));
#6090=DIRECTION('center_axis',(0.,0.,1.));
#6091=DIRECTION('ref_axis',(1.,0.,0.));
#6092=DIRECTION('center_axis',(0.,0.,1.));
#6093=DIRECTION('ref_axis',(1.,0.,0.));
#6094=DIRECTION('',(0.,0.,1.));
#6095=DIRECTION('center_axis',(0.,0.,1.));
#6096=DIRECTION('ref_axis',(1.,0.,0.));
#6097=DIRECTION('center_axis',(0.,0.,1.));
#6098=DIRECTION('ref_axis',(1.,0.,0.));
#6099=DIRECTION('',(0.,0.,1.));
#6100=DIRECTION('center_axis',(0.,1.,0.));
#6101=DIRECTION('ref_axis',(1.,0.,0.));
#6102=DIRECTION('center_axis',(0.,1.,0.));
#6103=DIRECTION('ref_axis',(1.,0.,0.));
#6104=DIRECTION('',(0.,1.,0.));
#6105=DIRECTION('center_axis',(0.,-1.,0.));
#6106=DIRECTION('ref_axis',(1.,0.,0.));
#6107=DIRECTION('center_axis',(0.,-1.,0.));
#6108=DIRECTION('ref_axis',(0.,0.,-1.));
#6109=DIRECTION('',(0.,0.,-1.));
#6110=DIRECTION('',(1.,0.,0.));
#6111=DIRECTION('',(0.,0.,1.));
#6112=DIRECTION('',(0.,0.,1.));
#6113=DIRECTION('',(-1.,0.,0.));
#6114=DIRECTION('',(0.,0.,-1.));
#6115=DIRECTION('',(-1.,0.,0.));
#6116=DIRECTION('',(0.,0.,1.));
#6117=DIRECTION('',(-1.,0.,0.));
#6118=DIRECTION('center_axis',(-1.,0.,0.));
#6119=DIRECTION('ref_axis',(0.,0.,1.));
#6120=DIRECTION('',(0.,0.,1.));
#6121=DIRECTION('',(0.,1.,0.));
#6122=DIRECTION('center_axis',(0.,0.,-1.));
#6123=DIRECTION('ref_axis',(-1.,0.,0.));
#6124=DIRECTION('',(-1.,0.,0.));
#6125=DIRECTION('',(0.,1.,0.));
#6126=DIRECTION('center_axis',(1.,0.,0.));
#6127=DIRECTION('ref_axis',(0.,0.,-1.));
#6128=DIRECTION('',(0.,0.,-1.));
#6129=DIRECTION('center_axis',(1.,0.,0.));
#6130=DIRECTION('ref_axis',(0.,0.,-1.));
#6131=DIRECTION('',(0.,0.,-1.));
#6132=DIRECTION('',(0.,1.,0.));
#6133=DIRECTION('center_axis',(0.,0.,1.));
#6134=DIRECTION('ref_axis',(1.,0.,0.));
#6135=DIRECTION('',(1.,0.,0.));
#6136=DIRECTION('',(0.,1.,0.));
#6137=DIRECTION('center_axis',(-1.,0.,0.));
#6138=DIRECTION('ref_axis',(0.,0.,1.));
#6139=DIRECTION('',(0.,0.,1.));
#6140=DIRECTION('',(0.,1.,0.));
#6141=DIRECTION('center_axis',(0.,0.,1.));
#6142=DIRECTION('ref_axis',(1.,0.,0.));
#6143=DIRECTION('',(1.,0.,0.));
#6144=DIRECTION('',(0.,1.,0.));
#6145=DIRECTION('center_axis',(1.,0.,0.));
#6146=DIRECTION('ref_axis',(0.,0.,-1.));
#6147=DIRECTION('',(0.,0.,-1.));
#6148=DIRECTION('',(0.,1.,0.));
#6149=DIRECTION('center_axis',(0.,0.,1.));
#6150=DIRECTION('ref_axis',(1.,0.,0.));
#6151=DIRECTION('',(1.,0.,0.));
#6152=DIRECTION('center_axis',(0.,1.,0.));
#6153=DIRECTION('ref_axis',(0.,0.,1.));
#7548=CARTESIAN_POINT('',(0.,0.,0.));
#7549=CARTESIAN_POINT('Origin',(-1.6,0.,1.3));
#7550=CARTESIAN_POINT('',(-1.2,0.340036762718386,1.3));
#7551=CARTESIAN_POINT('',(-1.2,-0.340036762718386,1.3));
#7552=CARTESIAN_POINT('',(-1.2,0.,1.3));
#7553=CARTESIAN_POINT('Origin',(-1.6,0.,1.3));
#7554=CARTESIAN_POINT('Origin',(-1.6,0.,0.6));
#7555=CARTESIAN_POINT('',(-1.2,0.340036762718386,0.6));
#7556=CARTESIAN_POINT('',(-1.2,0.340036762718386,0.6));
#7557=CARTESIAN_POINT('',(-1.2,-0.340036762718386,0.6));
#7558=CARTESIAN_POINT('Origin',(-1.6,0.,0.6));
#7559=CARTESIAN_POINT('',(-1.2,-0.340036762718386,0.6));
#7560=CARTESIAN_POINT('Origin',(1.6,0.,0.6));
#7561=CARTESIAN_POINT('',(1.2,0.340036762718386,1.3));
#7562=CARTESIAN_POINT('',(1.2,0.340036762718386,0.6));
#7563=CARTESIAN_POINT('',(1.2,0.340036762718386,0.6));
#7564=CARTESIAN_POINT('',(1.2,-0.340036762718386,1.3));
#7565=CARTESIAN_POINT('Origin',(1.6,0.,1.3));
#7566=CARTESIAN_POINT('',(1.2,-0.340036762718386,0.6));
#7567=CARTESIAN_POINT('',(1.2,-0.340036762718386,0.6));
#7568=CARTESIAN_POINT('Origin',(1.6,0.,0.6));
#7569=CARTESIAN_POINT('Origin',(1.6,0.,1.3));
#7570=CARTESIAN_POINT('',(1.2,0.,1.3));
#7571=CARTESIAN_POINT('Origin',(-2.1,0.,0.6));
#7572=CARTESIAN_POINT('',(-1.2,0.7,0.6));
#7573=CARTESIAN_POINT('',(-1.2,0.,0.6));
#7574=CARTESIAN_POINT('',(-2.1,0.7,0.6));
#7575=CARTESIAN_POINT('',(-1.2,0.7,0.6));
#7576=CARTESIAN_POINT('',(-2.1,-0.7,0.6));
#7577=CARTESIAN_POINT('',(-2.1,0.,0.6));
#7578=CARTESIAN_POINT('',(-1.2,-0.7,0.6));
#7579=CARTESIAN_POINT('',(-1.2,-0.7,0.6));
#7580=CARTESIAN_POINT('',(-1.2,0.,0.6));
#7581=CARTESIAN_POINT('',(-1.875,3.36777869765522E-17,0.6));
#7582=CARTESIAN_POINT('Origin',(-1.6,0.,0.6));
#7583=CARTESIAN_POINT('Origin',(-1.2,0.,0.6));
#7584=CARTESIAN_POINT('',(-1.2,-0.7,3.75));
#7585=CARTESIAN_POINT('',(-1.2,-0.7,3.75));
#7586=CARTESIAN_POINT('',(-1.2,0.7,3.75));
#7587=CARTESIAN_POINT('',(-1.2,0.,3.75));
#7588=CARTESIAN_POINT('',(-1.2,0.7,3.75));
#7589=CARTESIAN_POINT('',(-1.2,-2.02066721859313E-17,3.515));
#7590=CARTESIAN_POINT('Origin',(-1.2,0.,3.35));
#7591=CARTESIAN_POINT('Origin',(1.2,0.,0.6));
#7592=CARTESIAN_POINT('',(2.1,-0.7,0.6));
#7593=CARTESIAN_POINT('',(2.1,0.7,0.6));
#7594=CARTESIAN_POINT('',(2.1,0.,0.6));
#7595=CARTESIAN_POINT('',(1.2,0.7,0.6));
#7596=CARTESIAN_POINT('',(2.1,0.7,0.6));
#7597=CARTESIAN_POINT('',(1.2,0.,0.6));
#7598=CARTESIAN_POINT('',(1.2,-0.7,0.6));
#7599=CARTESIAN_POINT('',(1.2,0.,0.6));
#7600=CARTESIAN_POINT('',(2.1,-0.7,0.6));
#7601=CARTESIAN_POINT('',(1.325,3.36777869765522E-17,0.6));
#7602=CARTESIAN_POINT('Origin',(1.6,0.,0.6));
#7603=CARTESIAN_POINT('Origin',(0.1,0.,3.35));
#7604=CARTESIAN_POINT('',(0.1,-2.75545529808155E-17,3.575));
#7605=CARTESIAN_POINT('Origin',(0.1,0.,3.35));
#7606=CARTESIAN_POINT('',(1.2,2.75545529808155E-17,3.575));
#7607=CARTESIAN_POINT('',(0.1,-2.75545529808155E-17,3.575));
#7608=CARTESIAN_POINT('Origin',(1.2,0.,3.35));
#7609=CARTESIAN_POINT('Origin',(0.,0.,3.35));
#7610=CARTESIAN_POINT('',(-0.1,2.02066721859313E-17,3.515));
#7611=CARTESIAN_POINT('',(0.,-2.02066721859313E-17,3.515));
#7612=CARTESIAN_POINT('Origin',(-0.1,0.,3.35));
#7613=CARTESIAN_POINT('Origin',(-1.6,0.,-0.05));
#7614=CARTESIAN_POINT('',(-1.875,-3.36777869765522E-17,0.));
#7615=CARTESIAN_POINT('Origin',(-1.6,0.,0.));
#7616=CARTESIAN_POINT('',(-1.875,-3.36777869765522E-17,-0.05));
#7617=CARTESIAN_POINT('Origin',(1.6,0.,-0.05));
#7618=CARTESIAN_POINT('',(1.325,-3.36777869765522E-17,0.));
#7619=CARTESIAN_POINT('Origin',(1.6,0.,0.));
#7620=CARTESIAN_POINT('',(1.325,-3.36777869765522E-17,-0.05));
#7621=CARTESIAN_POINT('Origin',(0.,0.,2.3));
#7622=CARTESIAN_POINT('',(-0.6,-0.7,2.3));
#7623=CARTESIAN_POINT('Origin',(0.,-0.7,2.3));
#7624=CARTESIAN_POINT('',(-0.6,0.7,2.3));
#7625=CARTESIAN_POINT('',(-0.6,0.,2.3));
#7626=CARTESIAN_POINT('Origin',(0.,0.7,2.3));
#7627=CARTESIAN_POINT('Origin',(0.,-0.7,1.875));
#7628=CARTESIAN_POINT('',(-2.1,-0.7,0.));
#7629=CARTESIAN_POINT('',(-2.1,-0.7,0.6));
#7630=CARTESIAN_POINT('',(2.1,-0.7,0.));
#7631=CARTESIAN_POINT('',(-2.1,-0.7,0.));
#7632=CARTESIAN_POINT('',(2.1,-0.7,0.));
#7633=CARTESIAN_POINT('',(1.2,-0.7,3.75));
#7634=CARTESIAN_POINT('',(1.2,-0.7,0.6));
#7635=CARTESIAN_POINT('',(0.1,-0.7,3.75));
#7636=CARTESIAN_POINT('',(1.2,-0.7,3.75));
#7637=CARTESIAN_POINT('',(0.1,-0.7,2.95));
#7638=CARTESIAN_POINT('',(0.1,-0.7,3.75));
#7639=CARTESIAN_POINT('',(-0.1,-0.7,2.95));
#7640=CARTESIAN_POINT('',(0.1,-0.7,2.95));
#7641=CARTESIAN_POINT('',(-0.1,-0.7,3.75));
#7642=CARTESIAN_POINT('',(-0.1,-0.7,2.95));
#7643=CARTESIAN_POINT('',(-0.1,-0.7,3.75));
#7644=CARTESIAN_POINT('Origin',(-2.1,0.,0.));
#7645=CARTESIAN_POINT('',(-2.1,0.7,0.));
#7646=CARTESIAN_POINT('',(-2.1,0.7,0.6));
#7647=CARTESIAN_POINT('',(-2.1,0.,0.));
#7648=CARTESIAN_POINT('Origin',(2.1,0.,0.));
#7649=CARTESIAN_POINT('',(2.1,0.7,0.));
#7650=CARTESIAN_POINT('',(-2.1,0.7,0.));
#7651=CARTESIAN_POINT('',(2.1,0.,0.));
#7652=CARTESIAN_POINT('Origin',(2.1,0.,0.6));
#7653=CARTESIAN_POINT('',(2.1,0.7,0.));
#7654=CARTESIAN_POINT('Origin',(1.2,0.,3.75));
#7655=CARTESIAN_POINT('',(1.2,0.7,3.75));
#7656=CARTESIAN_POINT('',(1.2,0.7,0.6));
#7657=CARTESIAN_POINT('',(1.2,0.,3.75));
#7658=CARTESIAN_POINT('Origin',(0.1,0.,3.75));
#7659=CARTESIAN_POINT('',(0.1,0.7,3.75));
#7660=CARTESIAN_POINT('',(1.2,0.7,3.75));
#7661=CARTESIAN_POINT('',(0.1,0.,3.75));
#7662=CARTESIAN_POINT('Origin',(0.1,0.,2.95));
#7663=CARTESIAN_POINT('',(0.1,0.7,2.95));
#7664=CARTESIAN_POINT('',(0.1,0.7,3.75));
#7665=CARTESIAN_POINT('',(0.1,0.,2.95));
#7666=CARTESIAN_POINT('Origin',(-0.1,0.,2.95));
#7667=CARTESIAN_POINT('',(-0.1,0.7,2.95));
#7668=CARTESIAN_POINT('',(0.1,0.7,2.95));
#7669=CARTESIAN_POINT('',(-0.1,0.,2.95));
#7670=CARTESIAN_POINT('Origin',(-0.1,0.,3.75));
#7671=CARTESIAN_POINT('',(-0.1,0.7,3.75));
#7672=CARTESIAN_POINT('',(-0.1,0.7,2.95));
#7673=CARTESIAN_POINT('',(-0.1,0.,3.75));
#7674=CARTESIAN_POINT('Origin',(-1.2,0.,3.75));
#7675=CARTESIAN_POINT('',(-0.1,0.7,3.75));
#7676=CARTESIAN_POINT('Origin',(0.,0.7,1.875));
#10241=UNCERTAINTY_MEASURE_WITH_UNIT(LENGTH_MEASURE(0.001),#10293,
'DISTANCE_ACCURACY_VALUE',
'Maximum model space distance between geometric entities at asserted c
onnectivities');
#10264=UNCERTAINTY_MEASURE_WITH_UNIT(LENGTH_MEASURE(0.001),#10293,
'DISTANCE_ACCURACY_VALUE',
'Maximum model space distance between geometric entities at asserted c
onnectivities');
#10269=(
GEOMETRIC_REPRESENTATION_CONTEXT(3)
GLOBAL_UNCERTAINTY_ASSIGNED_CONTEXT((#10241))
GLOBAL_UNIT_ASSIGNED_CONTEXT((#10293,#10295,#10296))
REPRESENTATION_CONTEXT('','3D')
);
#10292=(
GEOMETRIC_REPRESENTATION_CONTEXT(3)
GLOBAL_UNCERTAINTY_ASSIGNED_CONTEXT((#10264))
GLOBAL_UNIT_ASSIGNED_CONTEXT((#10293,#10295,#10296))
REPRESENTATION_CONTEXT('','3D')
);
#10293=(
LENGTH_UNIT()
NAMED_UNIT(*)
SI_UNIT(.CENTI.,.METRE.)
);
#10295=(
NAMED_UNIT(*)
PLANE_ANGLE_UNIT()
SI_UNIT($,.RADIAN.)
);
#10296=(
NAMED_UNIT(*)
SI_UNIT($,.STERADIAN.)
SOLID_ANGLE_UNIT()
);
#10301=SHAPE_DEFINITION_REPRESENTATION(#10328,#10417);
#10328=PRODUCT_DEFINITION_SHAPE('',$,#10445);
#10417=SHAPE_REPRESENTATION('',(#5356),#10269);
#10440=PRODUCT_DEFINITION_CONTEXT('part definition',#10523,'design');
#10445=PRODUCT_DEFINITION('Relieved shaft support',
'Relieved shaft support',#10472,#10440);
#10472=PRODUCT_DEFINITION_FORMATION('',$,#10529);
#10523=APPLICATION_CONTEXT(
'Core Data for Automotive Mechanical Design Process');
#10524=PRODUCT_CONTEXT('part definition',#10523,'mechanical');
#10529=PRODUCT('Relieved shaft support','Relieved shaft support',
'Relieved shaft support',(#10524));
#10622=COLOUR_RGB('Grey',0.48,0.52,0.57);
#10623=FILL_AREA_STYLE_COLOUR('',#10622);
#10624=FILL_AREA_STYLE('',(#10623));
#10625=SURFACE_STYLE_FILL_AREA(#10624);
#10626=SURFACE_SIDE_STYLE('',(#10625));
#10627=SURFACE_STYLE_USAGE(.BOTH.,#10626);
#10628=PRESENTATION_STYLE_ASSIGNMENT((#10627));
ENDSEC;
END-ISO-10303-21;
